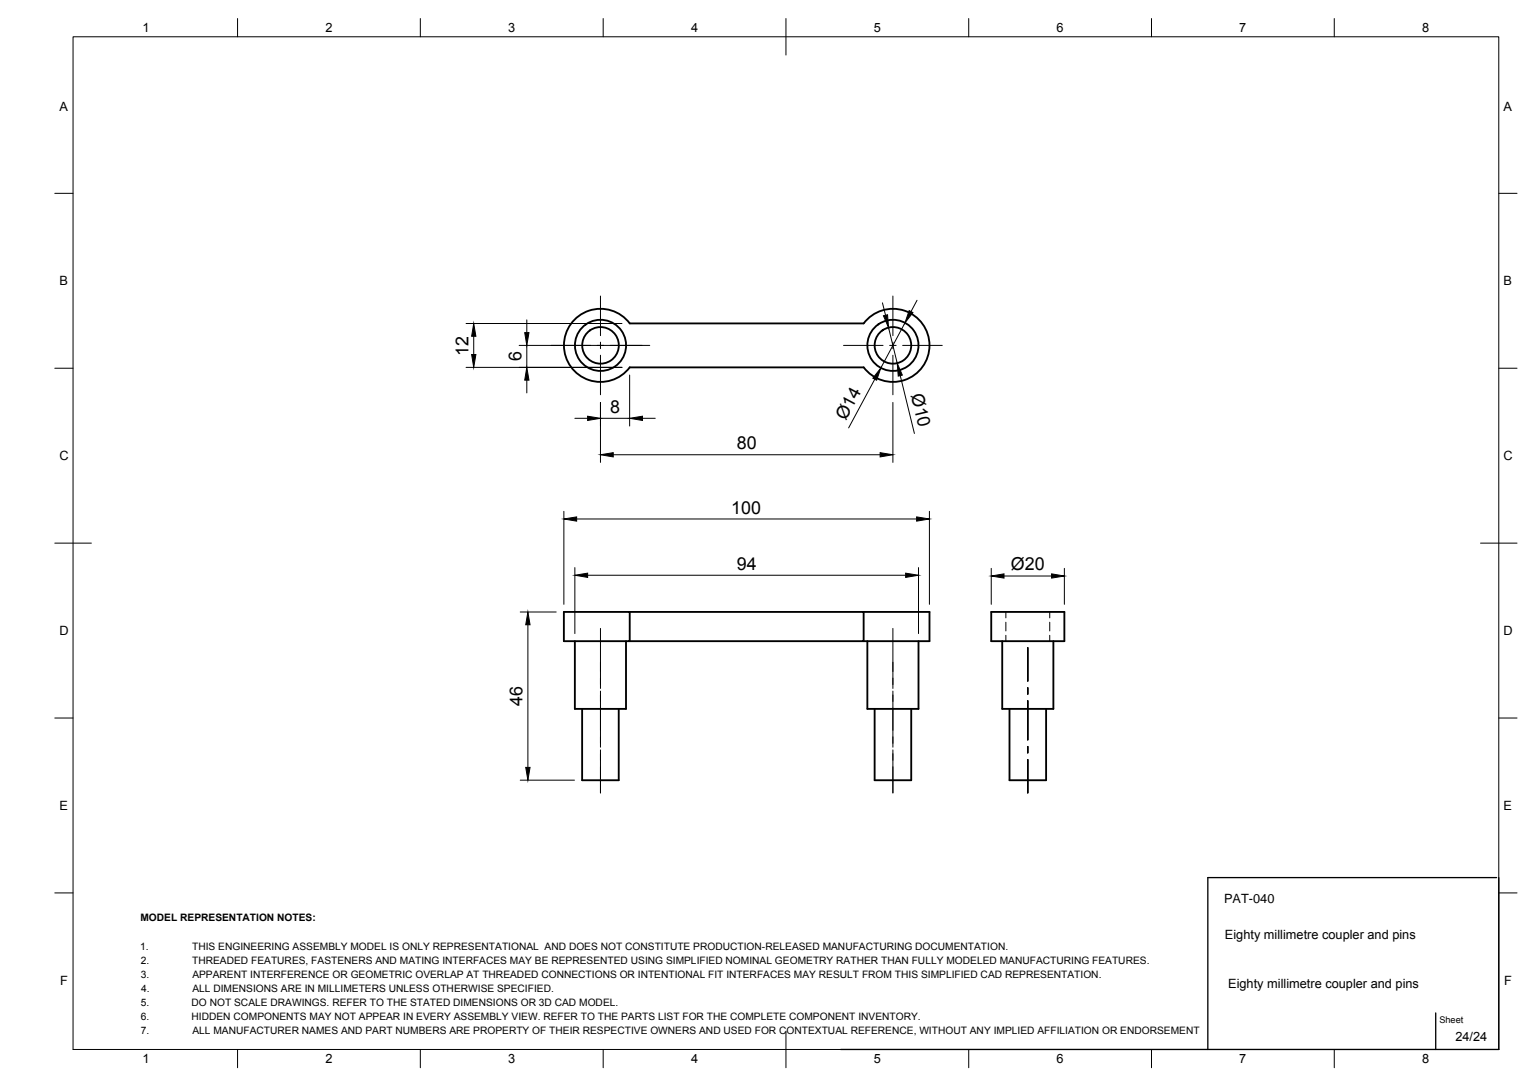
ISO-10303-21;
HEADER;
/* Generated by software containing ST-Developer
 * from STEP Tools, Inc. (www.steptools.com) 
 */

FILE_DESCRIPTION(
/* description */ ('Four-bar tabletop demonstrator'),
/* implementation_level */ '2;1');

FILE_NAME(
/* name */ 'Eighty millimetre coupler and pins.step',
/* time_stamp */ '2026-10-29T17:05:23-07:00',
/* author */ (''),
/* organization */ (''),
/* preprocessor_version */ 'ST-DEVELOPER v20.2',
/* originating_system */ 'Autodesk Translation Framework v15.17.0.0',
/* authorisation */ '');

FILE_SCHEMA (('AUTOMOTIVE_DESIGN { 1 0 10303 214 3 1 1 }'));
ENDSEC;

DATA;
#10=MECHANICAL_DESIGN_GEOMETRIC_PRESENTATION_REPRESENTATION('',(#356),#6705);
#318=SHAPE_REPRESENTATION_RELATIONSHIP('SRR','None',#6828,#333);
#333=ADVANCED_BREP_SHAPE_REPRESENTATION('',(#377),#6701);
#356=STYLED_ITEM('',(#6982),#377);
#377=MANIFOLD_SOLID_BREP('Body1',#3402);
#451=FACE_BOUND('',#1005,.T.);
#452=FACE_BOUND('',#1006,.T.);
#453=FACE_BOUND('',#1008,.T.);
#454=FACE_BOUND('',#1015,.T.);
#539=PLANE('',#3974);
#540=PLANE('',#3975);
#541=PLANE('',#3979);
#542=PLANE('',#3985);
#543=PLANE('',#3986);
#544=PLANE('',#3989);
#545=PLANE('',#3995);
#546=PLANE('',#3996);
#729=FACE_OUTER_BOUND('',#1002,.T.);
#730=FACE_OUTER_BOUND('',#1003,.T.);
#731=FACE_OUTER_BOUND('',#1004,.T.);
#732=FACE_OUTER_BOUND('',#1007,.T.);
#733=FACE_OUTER_BOUND('',#1009,.T.);
#734=FACE_OUTER_BOUND('',#1010,.T.);
#735=FACE_OUTER_BOUND('',#1011,.T.);
#736=FACE_OUTER_BOUND('',#1012,.T.);
#737=FACE_OUTER_BOUND('',#1013,.T.);
#738=FACE_OUTER_BOUND('',#1014,.T.);
#739=FACE_OUTER_BOUND('',#1016,.T.);
#740=FACE_OUTER_BOUND('',#1017,.T.);
#741=FACE_OUTER_BOUND('',#1018,.T.);
#742=FACE_OUTER_BOUND('',#1019,.T.);
#1002=EDGE_LOOP('',(#2966,#2967,#2968,#2969));
#1003=EDGE_LOOP('',(#2970,#2971,#2972,#2973));
#1004=EDGE_LOOP('',(#2974,#2975,#2976,#2977));
#1005=EDGE_LOOP('',(#2978));
#1006=EDGE_LOOP('',(#2979));
#1007=EDGE_LOOP('',(#2980));
#1008=EDGE_LOOP('',(#2981));
#1009=EDGE_LOOP('',(#2982,#2983,#2984,#2985));
#1010=EDGE_LOOP('',(#2986,#2987,#2988,#2989));
#1011=EDGE_LOOP('',(#2990));
#1012=EDGE_LOOP('',(#2991,#2992,#2993,#2994));
#1013=EDGE_LOOP('',(#2995,#2996,#2997,#2998));
#1014=EDGE_LOOP('',(#2999));
#1015=EDGE_LOOP('',(#3000));
#1016=EDGE_LOOP('',(#3001,#3002,#3003,#3004));
#1017=EDGE_LOOP('',(#3005,#3006,#3007,#3008));
#1018=EDGE_LOOP('',(#3009,#3010,#3011,#3012));
#1019=EDGE_LOOP('',(#3013));
#1180=LINE('',#6419,#1350);
#1181=LINE('',#6423,#1351);
#1182=LINE('',#6427,#1352);
#1183=LINE('',#6429,#1353);
#1184=LINE('',#6430,#1354);
#1185=LINE('',#6433,#1355);
#1186=LINE('',#6445,#1356);
#1187=LINE('',#6448,#1357);
#1188=LINE('',#6453,#1358);
#1189=LINE('',#6454,#1359);
#1190=LINE('',#6463,#1360);
#1191=LINE('',#6466,#1361);
#1350=VECTOR('',#4997,1.);
#1351=VECTOR('',#5000,1.);
#1352=VECTOR('',#5005,1.);
#1353=VECTOR('',#5006,1.);
#1354=VECTOR('',#5007,1.);
#1355=VECTOR('',#5010,1.);
#1356=VECTOR('',#5025,0.699999999999999);
#1357=VECTOR('',#5028,0.5);
#1358=VECTOR('',#5035,1.);
#1359=VECTOR('',#5036,1.);
#1360=VECTOR('',#5049,0.7);
#1361=VECTOR('',#5052,0.5);
#1575=CIRCLE('',#3972,1.);
#1576=CIRCLE('',#3973,1.);
#1577=CIRCLE('',#3976,1.);
#1578=CIRCLE('',#3977,0.699999999999999);
#1579=CIRCLE('',#3978,0.7);
#1580=CIRCLE('',#3980,0.699999999999999);
#1581=CIRCLE('',#3981,0.5);
#1582=CIRCLE('',#3984,0.5);
#1583=CIRCLE('',#3988,1.);
#1584=CIRCLE('',#3990,0.7);
#1585=CIRCLE('',#3991,0.5);
#1586=CIRCLE('',#3994,0.5);
#1834=VERTEX_POINT('',#6417);
#1835=VERTEX_POINT('',#6418);
#1836=VERTEX_POINT('',#6420);
#1837=VERTEX_POINT('',#6422);
#1838=VERTEX_POINT('',#6426);
#1839=VERTEX_POINT('',#6428);
#1840=VERTEX_POINT('',#6432);
#1841=VERTEX_POINT('',#6435);
#1842=VERTEX_POINT('',#6437);
#1843=VERTEX_POINT('',#6440);
#1844=VERTEX_POINT('',#6442);
#1845=VERTEX_POINT('',#6447);
#1846=VERTEX_POINT('',#6452);
#1847=VERTEX_POINT('',#6458);
#1848=VERTEX_POINT('',#6460);
#1849=VERTEX_POINT('',#6465);
#2219=EDGE_CURVE('',#1834,#1835,#1180,.T.);
#2220=EDGE_CURVE('',#1836,#1834,#1575,.T.);
#2221=EDGE_CURVE('',#1837,#1836,#1181,.T.);
#2222=EDGE_CURVE('',#1837,#1835,#1576,.T.);
#2223=EDGE_CURVE('',#1838,#1835,#1182,.T.);
#2224=EDGE_CURVE('',#1839,#1838,#1183,.T.);
#2225=EDGE_CURVE('',#1834,#1839,#1184,.T.);
#2226=EDGE_CURVE('',#1837,#1840,#1185,.T.);
#2227=EDGE_CURVE('',#1838,#1840,#1577,.T.);
#2228=EDGE_CURVE('',#1841,#1841,#1578,.T.);
#2229=EDGE_CURVE('',#1842,#1842,#1579,.T.);
#2230=EDGE_CURVE('',#1843,#1843,#1580,.T.);
#2231=EDGE_CURVE('',#1844,#1844,#1581,.T.);
#2232=EDGE_CURVE('',#1841,#1843,#1186,.T.);
#2233=EDGE_CURVE('',#1844,#1845,#1187,.T.);
#2234=EDGE_CURVE('',#1845,#1845,#1582,.T.);
#2235=EDGE_CURVE('',#1846,#1836,#1188,.T.);
#2236=EDGE_CURVE('',#1840,#1846,#1189,.T.);
#2237=EDGE_CURVE('',#1839,#1846,#1583,.T.);
#2238=EDGE_CURVE('',#1847,#1847,#1584,.T.);
#2239=EDGE_CURVE('',#1848,#1848,#1585,.T.);
#2240=EDGE_CURVE('',#1842,#1847,#1190,.T.);
#2241=EDGE_CURVE('',#1848,#1849,#1191,.T.);
#2242=EDGE_CURVE('',#1849,#1849,#1586,.T.);
#2966=ORIENTED_EDGE('',*,*,#2219,.F.);
#2967=ORIENTED_EDGE('',*,*,#2220,.F.);
#2968=ORIENTED_EDGE('',*,*,#2221,.F.);
#2969=ORIENTED_EDGE('',*,*,#2222,.T.);
#2970=ORIENTED_EDGE('',*,*,#2219,.T.);
#2971=ORIENTED_EDGE('',*,*,#2223,.F.);
#2972=ORIENTED_EDGE('',*,*,#2224,.F.);
#2973=ORIENTED_EDGE('',*,*,#2225,.F.);
#2974=ORIENTED_EDGE('',*,*,#2222,.F.);
#2975=ORIENTED_EDGE('',*,*,#2226,.T.);
#2976=ORIENTED_EDGE('',*,*,#2227,.F.);
#2977=ORIENTED_EDGE('',*,*,#2223,.T.);
#2978=ORIENTED_EDGE('',*,*,#2228,.T.);
#2979=ORIENTED_EDGE('',*,*,#2229,.T.);
#2980=ORIENTED_EDGE('',*,*,#2230,.F.);
#2981=ORIENTED_EDGE('',*,*,#2231,.F.);
#2982=ORIENTED_EDGE('',*,*,#2228,.F.);
#2983=ORIENTED_EDGE('',*,*,#2232,.T.);
#2984=ORIENTED_EDGE('',*,*,#2230,.T.);
#2985=ORIENTED_EDGE('',*,*,#2232,.F.);
#2986=ORIENTED_EDGE('',*,*,#2231,.T.);
#2987=ORIENTED_EDGE('',*,*,#2233,.T.);
#2988=ORIENTED_EDGE('',*,*,#2234,.T.);
#2989=ORIENTED_EDGE('',*,*,#2233,.F.);
#2990=ORIENTED_EDGE('',*,*,#2234,.F.);
#2991=ORIENTED_EDGE('',*,*,#2221,.T.);
#2992=ORIENTED_EDGE('',*,*,#2235,.F.);
#2993=ORIENTED_EDGE('',*,*,#2236,.F.);
#2994=ORIENTED_EDGE('',*,*,#2226,.F.);
#2995=ORIENTED_EDGE('',*,*,#2224,.T.);
#2996=ORIENTED_EDGE('',*,*,#2227,.T.);
#2997=ORIENTED_EDGE('',*,*,#2236,.T.);
#2998=ORIENTED_EDGE('',*,*,#2237,.F.);
#2999=ORIENTED_EDGE('',*,*,#2238,.F.);
#3000=ORIENTED_EDGE('',*,*,#2239,.F.);
#3001=ORIENTED_EDGE('',*,*,#2229,.F.);
#3002=ORIENTED_EDGE('',*,*,#2240,.T.);
#3003=ORIENTED_EDGE('',*,*,#2238,.T.);
#3004=ORIENTED_EDGE('',*,*,#2240,.F.);
#3005=ORIENTED_EDGE('',*,*,#2239,.T.);
#3006=ORIENTED_EDGE('',*,*,#2241,.T.);
#3007=ORIENTED_EDGE('',*,*,#2242,.T.);
#3008=ORIENTED_EDGE('',*,*,#2241,.F.);
#3009=ORIENTED_EDGE('',*,*,#2225,.T.);
#3010=ORIENTED_EDGE('',*,*,#2237,.T.);
#3011=ORIENTED_EDGE('',*,*,#2235,.T.);
#3012=ORIENTED_EDGE('',*,*,#2220,.T.);
#3013=ORIENTED_EDGE('',*,*,#2242,.F.);
#3166=CYLINDRICAL_SURFACE('',#3971,1.);
#3167=CYLINDRICAL_SURFACE('',#3982,0.699999999999999);
#3168=CYLINDRICAL_SURFACE('',#3983,0.5);
#3169=CYLINDRICAL_SURFACE('',#3987,1.);
#3170=CYLINDRICAL_SURFACE('',#3992,0.7);
#3171=CYLINDRICAL_SURFACE('',#3993,0.5);
#3345=ADVANCED_FACE('',(#729),#3166,.T.);
#3346=ADVANCED_FACE('',(#730),#539,.T.);
#3347=ADVANCED_FACE('',(#731,#451,#452),#540,.F.);
#3348=ADVANCED_FACE('',(#732,#453),#541,.F.);
#3349=ADVANCED_FACE('',(#733),#3167,.T.);
#3350=ADVANCED_FACE('',(#734),#3168,.T.);
#3351=ADVANCED_FACE('',(#735),#542,.F.);
#3352=ADVANCED_FACE('',(#736),#543,.T.);
#3353=ADVANCED_FACE('',(#737),#3169,.T.);
#3354=ADVANCED_FACE('',(#738,#454),#544,.F.);
#3355=ADVANCED_FACE('',(#739),#3170,.T.);
#3356=ADVANCED_FACE('',(#740),#3171,.T.);
#3357=ADVANCED_FACE('',(#741),#545,.T.);
#3358=ADVANCED_FACE('',(#742),#546,.F.);
#3402=CLOSED_SHELL('',(#3345,#3346,#3347,#3348,#3349,#3350,#3351,#3352,
#3353,#3354,#3355,#3356,#3357,#3358));
#3970=AXIS2_PLACEMENT_3D('',#6415,#4993,#4994);
#3971=AXIS2_PLACEMENT_3D('',#6416,#4995,#4996);
#3972=AXIS2_PLACEMENT_3D('',#6421,#4998,#4999);
#3973=AXIS2_PLACEMENT_3D('',#6424,#5001,#5002);
#3974=AXIS2_PLACEMENT_3D('',#6425,#5003,#5004);
#3975=AXIS2_PLACEMENT_3D('',#6431,#5008,#5009);
#3976=AXIS2_PLACEMENT_3D('',#6434,#5011,#5012);
#3977=AXIS2_PLACEMENT_3D('',#6436,#5013,#5014);
#3978=AXIS2_PLACEMENT_3D('',#6438,#5015,#5016);
#3979=AXIS2_PLACEMENT_3D('',#6439,#5017,#5018);
#3980=AXIS2_PLACEMENT_3D('',#6441,#5019,#5020);
#3981=AXIS2_PLACEMENT_3D('',#6443,#5021,#5022);
#3982=AXIS2_PLACEMENT_3D('',#6444,#5023,#5024);
#3983=AXIS2_PLACEMENT_3D('',#6446,#5026,#5027);
#3984=AXIS2_PLACEMENT_3D('',#6449,#5029,#5030);
#3985=AXIS2_PLACEMENT_3D('',#6450,#5031,#5032);
#3986=AXIS2_PLACEMENT_3D('',#6451,#5033,#5034);
#3987=AXIS2_PLACEMENT_3D('',#6455,#5037,#5038);
#3988=AXIS2_PLACEMENT_3D('',#6456,#5039,#5040);
#3989=AXIS2_PLACEMENT_3D('',#6457,#5041,#5042);
#3990=AXIS2_PLACEMENT_3D('',#6459,#5043,#5044);
#3991=AXIS2_PLACEMENT_3D('',#6461,#5045,#5046);
#3992=AXIS2_PLACEMENT_3D('',#6462,#5047,#5048);
#3993=AXIS2_PLACEMENT_3D('',#6464,#5050,#5051);
#3994=AXIS2_PLACEMENT_3D('',#6467,#5053,#5054);
#3995=AXIS2_PLACEMENT_3D('',#6468,#5055,#5056);
#3996=AXIS2_PLACEMENT_3D('',#6469,#5057,#5058);
#4993=DIRECTION('axis',(0.,0.,1.));
#4994=DIRECTION('refdir',(1.,0.,0.));
#4995=DIRECTION('center_axis',(0.,0.,1.));
#4996=DIRECTION('ref_axis',(1.,0.,0.));
#4997=DIRECTION('',(0.,0.,-1.));
#4998=DIRECTION('center_axis',(0.,0.,1.));
#4999=DIRECTION('ref_axis',(1.,0.,0.));
#5000=DIRECTION('',(0.,0.,1.));
#5001=DIRECTION('center_axis',(0.,0.,1.));
#5002=DIRECTION('ref_axis',(1.,0.,0.));
#5003=DIRECTION('center_axis',(0.,1.,0.));
#5004=DIRECTION('ref_axis',(-1.,0.,0.));
#5005=DIRECTION('',(1.,0.,0.));
#5006=DIRECTION('',(0.,0.,-1.));
#5007=DIRECTION('',(-1.,0.,0.));
#5008=DIRECTION('center_axis',(0.,0.,1.));
#5009=DIRECTION('ref_axis',(1.,0.,0.));
#5010=DIRECTION('',(-1.,0.,0.));
#5011=DIRECTION('center_axis',(0.,0.,1.));
#5012=DIRECTION('ref_axis',(1.,0.,0.));
#5013=DIRECTION('center_axis',(0.,0.,1.));
#5014=DIRECTION('ref_axis',(1.,0.,0.));
#5015=DIRECTION('center_axis',(0.,0.,1.));
#5016=DIRECTION('ref_axis',(1.,0.,0.));
#5017=DIRECTION('center_axis',(0.,0.,1.));
#5018=DIRECTION('ref_axis',(1.,0.,0.));
#5019=DIRECTION('center_axis',(0.,0.,1.));
#5020=DIRECTION('ref_axis',(1.,0.,0.));
#5021=DIRECTION('center_axis',(0.,0.,-1.));
#5022=DIRECTION('ref_axis',(1.,0.,0.));
#5023=DIRECTION('center_axis',(0.,0.,1.));
#5024=DIRECTION('ref_axis',(1.,0.,0.));
#5025=DIRECTION('',(0.,0.,-1.));
#5026=DIRECTION('center_axis',(0.,0.,1.));
#5027=DIRECTION('ref_axis',(1.,0.,0.));
#5028=DIRECTION('',(0.,0.,-1.));
#5029=DIRECTION('center_axis',(0.,0.,1.));
#5030=DIRECTION('ref_axis',(1.,0.,0.));
#5031=DIRECTION('center_axis',(0.,0.,1.));
#5032=DIRECTION('ref_axis',(1.,0.,0.));
#5033=DIRECTION('center_axis',(0.,-1.,0.));
#5034=DIRECTION('ref_axis',(1.,0.,0.));
#5035=DIRECTION('',(1.,0.,0.));
#5036=DIRECTION('',(0.,0.,1.));
#5037=DIRECTION('center_axis',(0.,0.,1.));
#5038=DIRECTION('ref_axis',(-1.,1.22464679914735E-16,0.));
#5039=DIRECTION('center_axis',(0.,0.,1.));
#5040=DIRECTION('ref_axis',(1.,0.,0.));
#5041=DIRECTION('center_axis',(0.,0.,1.));
#5042=DIRECTION('ref_axis',(1.,0.,0.));
#5043=DIRECTION('center_axis',(0.,0.,1.));
#5044=DIRECTION('ref_axis',(1.,0.,0.));
#5045=DIRECTION('center_axis',(0.,0.,-1.));
#5046=DIRECTION('ref_axis',(1.,0.,0.));
#5047=DIRECTION('center_axis',(0.,0.,1.));
#5048=DIRECTION('ref_axis',(1.,0.,0.));
#5049=DIRECTION('',(0.,0.,-1.));
#5050=DIRECTION('center_axis',(0.,0.,1.));
#5051=DIRECTION('ref_axis',(1.,0.,0.));
#5052=DIRECTION('',(0.,0.,-1.));
#5053=DIRECTION('center_axis',(0.,0.,1.));
#5054=DIRECTION('ref_axis',(1.,0.,0.));
#5055=DIRECTION('center_axis',(0.,0.,1.));
#5056=DIRECTION('ref_axis',(1.,0.,0.));
#5057=DIRECTION('center_axis',(0.,0.,1.));
#5058=DIRECTION('ref_axis',(1.,0.,0.));
#6415=CARTESIAN_POINT('',(0.,0.,0.));
#6416=CARTESIAN_POINT('Origin',(10.,3.46410161513775,7.55));
#6417=CARTESIAN_POINT('',(9.2,4.06410161513775,8.35));
#6418=CARTESIAN_POINT('',(9.2,4.06410161513775,7.55));
#6419=CARTESIAN_POINT('',(9.2,4.06410161513775,7.55));
#6420=CARTESIAN_POINT('',(9.2,2.86410161513775,8.35));
#6421=CARTESIAN_POINT('Origin',(10.,3.46410161513775,8.35));
#6422=CARTESIAN_POINT('',(9.2,2.86410161513775,7.55));
#6423=CARTESIAN_POINT('',(9.2,2.86410161513775,7.55));
#6424=CARTESIAN_POINT('Origin',(10.,3.46410161513775,7.55));
#6425=CARTESIAN_POINT('Origin',(10.,4.06410161513775,7.55));
#6426=CARTESIAN_POINT('',(2.8,4.06410161513775,7.55));
#6427=CARTESIAN_POINT('',(2.,4.06410161513775,7.55));
#6428=CARTESIAN_POINT('',(2.8,4.06410161513775,8.35));
#6429=CARTESIAN_POINT('',(2.8,4.06410161513775,7.55));
#6430=CARTESIAN_POINT('',(2.,4.06410161513775,8.35));
#6431=CARTESIAN_POINT('Origin',(2.,3.46410161513775,7.55));
#6432=CARTESIAN_POINT('',(2.8,2.86410161513775,7.55));
#6433=CARTESIAN_POINT('',(10.,2.86410161513775,7.55));
#6434=CARTESIAN_POINT('Origin',(2.,3.46410161513775,7.55));
#6435=CARTESIAN_POINT('',(9.3,3.46410161513775,7.55));
#6436=CARTESIAN_POINT('Origin',(10.,3.46410161513775,7.55));
#6437=CARTESIAN_POINT('',(1.3,3.46410161513775,7.55));
#6438=CARTESIAN_POINT('Origin',(2.,3.46410161513775,7.55));
#6439=CARTESIAN_POINT('Origin',(10.,3.46410161513775,5.7));
#6440=CARTESIAN_POINT('',(9.3,3.46410161513775,5.7));
#6441=CARTESIAN_POINT('Origin',(10.,3.46410161513775,5.7));
#6442=CARTESIAN_POINT('',(9.5,3.46410161513775,5.7));
#6443=CARTESIAN_POINT('Origin',(10.,3.46410161513775,5.7));
#6444=CARTESIAN_POINT('Origin',(10.,3.46410161513775,5.7));
#6445=CARTESIAN_POINT('',(9.3,3.46410161513775,5.7));
#6446=CARTESIAN_POINT('Origin',(10.,3.46410161513775,3.75));
#6447=CARTESIAN_POINT('',(9.5,3.46410161513775,3.75));
#6448=CARTESIAN_POINT('',(9.5,3.46410161513775,3.75));
#6449=CARTESIAN_POINT('Origin',(10.,3.46410161513775,3.75));
#6450=CARTESIAN_POINT('Origin',(10.,3.46410161513775,3.75));
#6451=CARTESIAN_POINT('Origin',(2.,2.86410161513775,7.55));
#6452=CARTESIAN_POINT('',(2.8,2.86410161513775,8.35));
#6453=CARTESIAN_POINT('',(10.,2.86410161513775,8.35));
#6454=CARTESIAN_POINT('',(2.8,2.86410161513775,7.55));
#6455=CARTESIAN_POINT('Origin',(2.,3.46410161513775,7.55));
#6456=CARTESIAN_POINT('Origin',(2.,3.46410161513775,8.35));
#6457=CARTESIAN_POINT('Origin',(2.,3.46410161513775,5.7));
#6458=CARTESIAN_POINT('',(1.3,3.46410161513775,5.7));
#6459=CARTESIAN_POINT('Origin',(2.,3.46410161513775,5.7));
#6460=CARTESIAN_POINT('',(1.5,3.46410161513775,5.7));
#6461=CARTESIAN_POINT('Origin',(2.,3.46410161513775,5.7));
#6462=CARTESIAN_POINT('Origin',(2.,3.46410161513775,5.7));
#6463=CARTESIAN_POINT('',(1.3,3.46410161513775,5.7));
#6464=CARTESIAN_POINT('Origin',(2.,3.46410161513775,3.75));
#6465=CARTESIAN_POINT('',(1.5,3.46410161513775,3.75));
#6466=CARTESIAN_POINT('',(1.5,3.46410161513775,3.75));
#6467=CARTESIAN_POINT('Origin',(2.,3.46410161513775,3.75));
#6468=CARTESIAN_POINT('Origin',(2.,3.46410161513775,8.35));
#6469=CARTESIAN_POINT('Origin',(2.,3.46410161513775,3.75));
#6679=UNCERTAINTY_MEASURE_WITH_UNIT(LENGTH_MEASURE(0.001),#6706,
'DISTANCE_ACCURACY_VALUE',
'Maximum model space distance between geometric entities at asserted c
onnectivities');
#6683=UNCERTAINTY_MEASURE_WITH_UNIT(LENGTH_MEASURE(0.001),#6706,
'DISTANCE_ACCURACY_VALUE',
'Maximum model space distance between geometric entities at asserted c
onnectivities');
#6701=(
GEOMETRIC_REPRESENTATION_CONTEXT(3)
GLOBAL_UNCERTAINTY_ASSIGNED_CONTEXT((#6679))
GLOBAL_UNIT_ASSIGNED_CONTEXT((#6706,#6708,#6709))
REPRESENTATION_CONTEXT('','3D')
);
#6705=(
GEOMETRIC_REPRESENTATION_CONTEXT(3)
GLOBAL_UNCERTAINTY_ASSIGNED_CONTEXT((#6683))
GLOBAL_UNIT_ASSIGNED_CONTEXT((#6706,#6708,#6709))
REPRESENTATION_CONTEXT('','3D')
);
#6706=(
LENGTH_UNIT()
NAMED_UNIT(*)
SI_UNIT(.CENTI.,.METRE.)
);
#6708=(
NAMED_UNIT(*)
PLANE_ANGLE_UNIT()
SI_UNIT($,.RADIAN.)
);
#6709=(
NAMED_UNIT(*)
SI_UNIT($,.STERADIAN.)
SOLID_ANGLE_UNIT()
);
#6727=SHAPE_DEFINITION_REPRESENTATION(#6776,#6828);
#6776=PRODUCT_DEFINITION_SHAPE('',$,#6850);
#6828=SHAPE_REPRESENTATION('',(#3970),#6701);
#6832=PRODUCT_DEFINITION_CONTEXT('part definition',#6897,'design');
#6850=PRODUCT_DEFINITION('Eighty millimetre coupler and pins',
'Eighty millimetre coupler and pins',#6871,#6832);
#6871=PRODUCT_DEFINITION_FORMATION('',$,#6916);
#6897=APPLICATION_CONTEXT(
'Core Data for Automotive Mechanical Design Process');
#6898=PRODUCT_CONTEXT('part definition',#6897,'mechanical');
#6916=PRODUCT('Eighty millimetre coupler and pins',
'Eighty millimetre coupler and pins',
'Eighty millimetre coupler and pins',(#6898));
#6976=COLOUR_RGB('Sky Blue',0.24,0.69,0.87);
#6977=FILL_AREA_STYLE_COLOUR('',#6976);
#6978=FILL_AREA_STYLE('',(#6977));
#6979=SURFACE_STYLE_FILL_AREA(#6978);
#6980=SURFACE_SIDE_STYLE('',(#6979));
#6981=SURFACE_STYLE_USAGE(.BOTH.,#6980);
#6982=PRESENTATION_STYLE_ASSIGNMENT((#6981));
ENDSEC;
END-ISO-10303-21;
